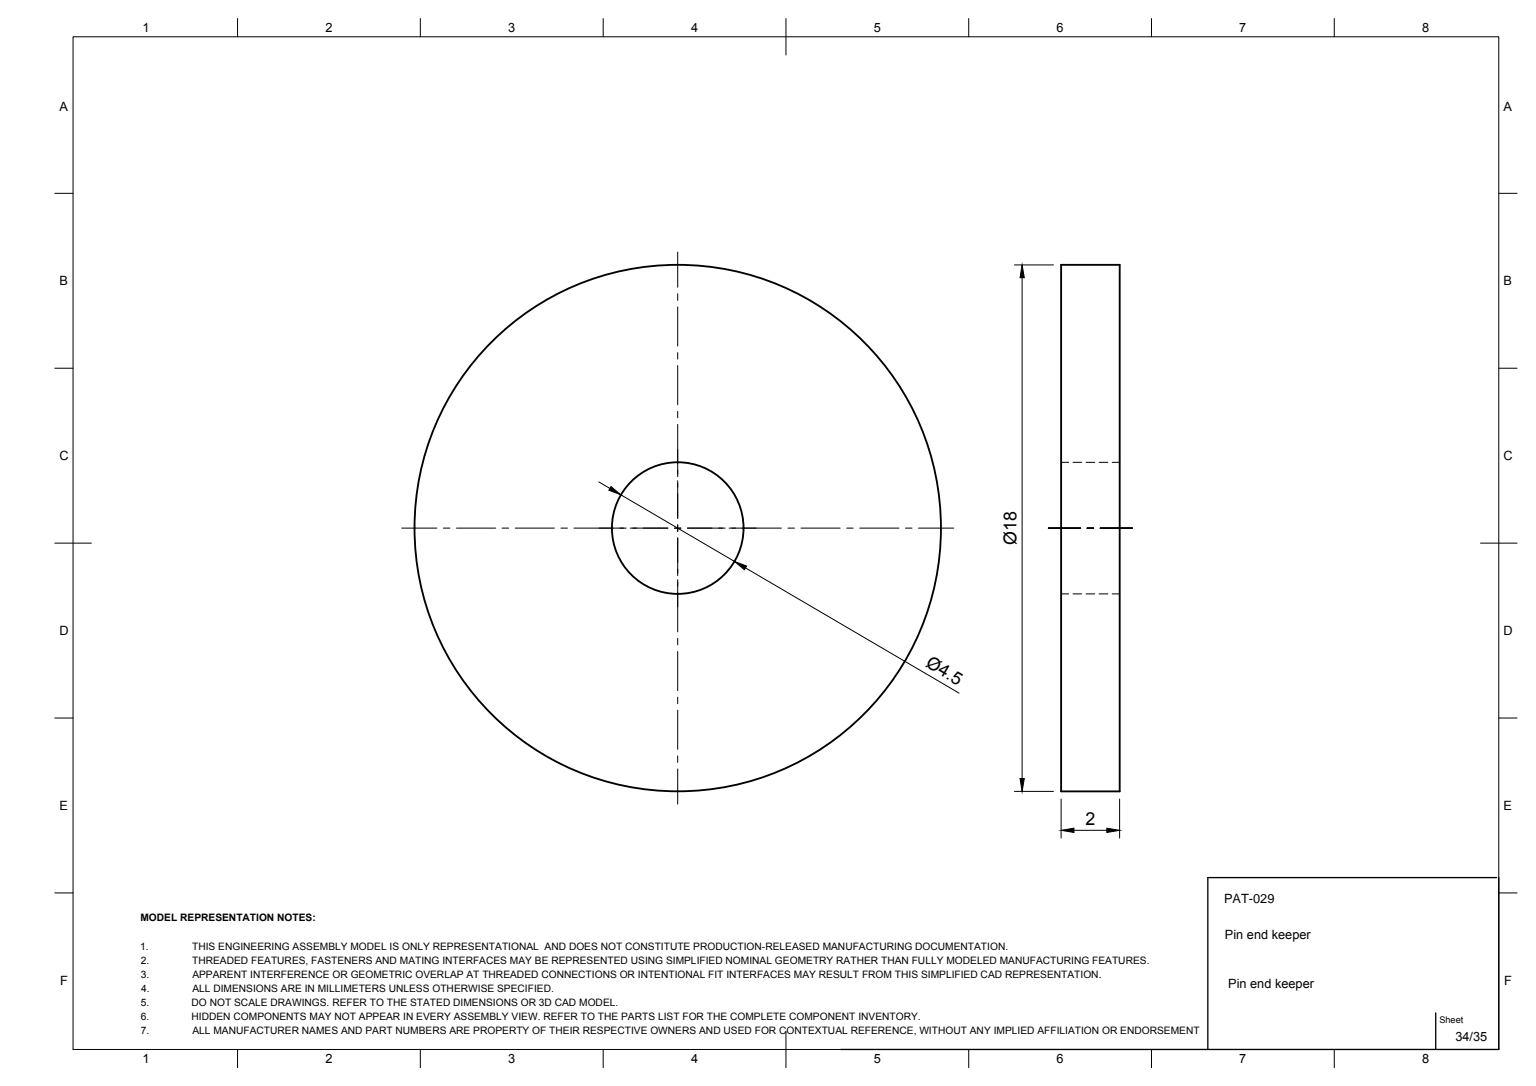
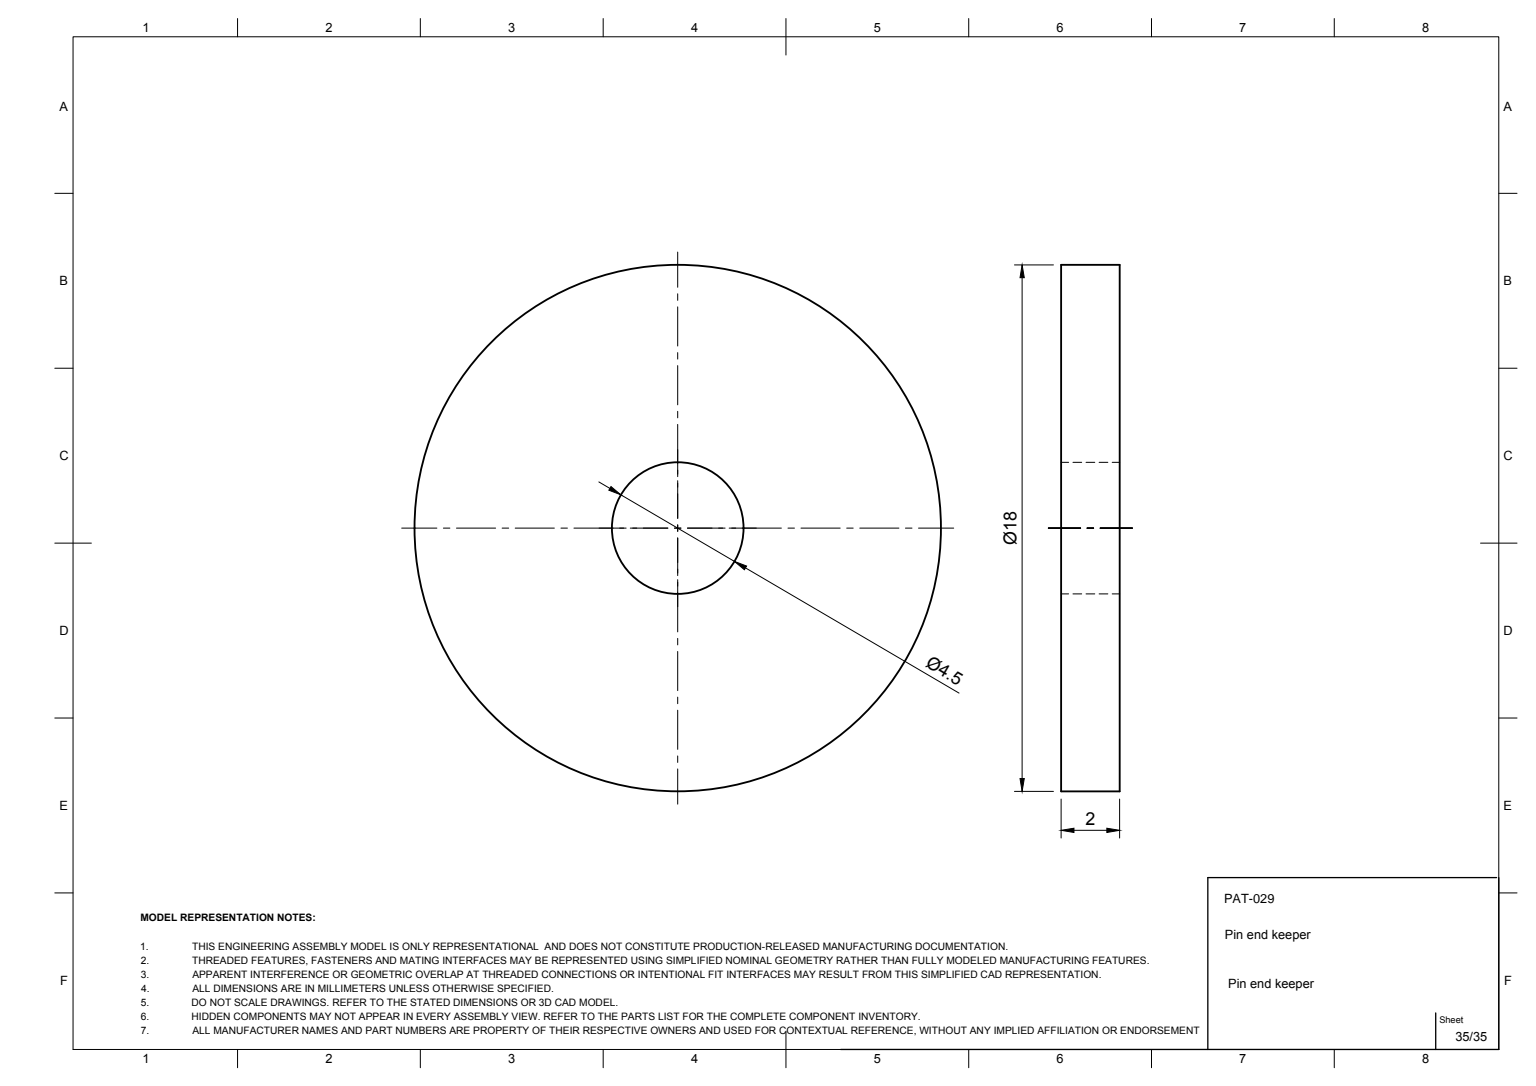
ISO-10303-21;
HEADER;
/* Generated by software containing ST-Developer
 * from STEP Tools, Inc. (www.steptools.com) 
 */

FILE_DESCRIPTION(
/* description */ ('Door-style hinge test fixture with detent'),
/* implementation_level */ '2;1');

FILE_NAME(
/* name */ 'Pin end keeper.step',
/* time_stamp */ '2026-10-28T03:24:57-07:00',
/* author */ (''),
/* organization */ (''),
/* preprocessor_version */ 'ST-DEVELOPER v20.2',
/* originating_system */ 'Autodesk Translation Framework v15.17.0.0',
/* authorisation */ '');

FILE_SCHEMA (('AUTOMOTIVE_DESIGN { 1 0 10303 214 3 1 1 }'));
ENDSEC;

DATA;
#10=MECHANICAL_DESIGN_GEOMETRIC_PRESENTATION_REPRESENTATION('',(#359),#9813);
#288=SHAPE_REPRESENTATION_RELATIONSHIP('SRR','None',#9967,#319);
#319=ADVANCED_BREP_SHAPE_REPRESENTATION('',(#397),#9810);
#359=STYLED_ITEM('',(#10183),#397);
#397=MANIFOLD_SOLID_BREP('Body1',#4792);
#495=FACE_BOUND('',#1307,.T.);
#496=FACE_BOUND('',#1309,.T.);
#648=PLANE('',#5705);
#649=PLANE('',#5706);
#923=FACE_OUTER_BOUND('',#1304,.T.);
#924=FACE_OUTER_BOUND('',#1305,.T.);
#925=FACE_OUTER_BOUND('',#1306,.T.);
#926=FACE_OUTER_BOUND('',#1308,.T.);
#1304=EDGE_LOOP('',(#4293,#4294,#4295,#4296));
#1305=EDGE_LOOP('',(#4297,#4298,#4299,#4300));
#1306=EDGE_LOOP('',(#4301));
#1307=EDGE_LOOP('',(#4302));
#1308=EDGE_LOOP('',(#4303));
#1309=EDGE_LOOP('',(#4304));
#1626=LINE('',#9638,#1946);
#1627=LINE('',#9644,#1947);
#1946=VECTOR('',#7169,0.225);
#1947=VECTOR('',#7176,0.9);
#2205=CIRCLE('',#5700,0.225);
#2206=CIRCLE('',#5701,0.225);
#2207=CIRCLE('',#5703,0.9);
#2208=CIRCLE('',#5704,0.9);
#2592=VERTEX_POINT('',#9635);
#2593=VERTEX_POINT('',#9637);
#2594=VERTEX_POINT('',#9641);
#2595=VERTEX_POINT('',#9643);
#3163=EDGE_CURVE('',#2592,#2592,#2205,.T.);
#3164=EDGE_CURVE('',#2592,#2593,#1626,.T.);
#3165=EDGE_CURVE('',#2593,#2593,#2206,.T.);
#3166=EDGE_CURVE('',#2594,#2594,#2207,.T.);
#3167=EDGE_CURVE('',#2594,#2595,#1627,.T.);
#3168=EDGE_CURVE('',#2595,#2595,#2208,.T.);
#4293=ORIENTED_EDGE('',*,*,#3163,.F.);
#4294=ORIENTED_EDGE('',*,*,#3164,.T.);
#4295=ORIENTED_EDGE('',*,*,#3165,.T.);
#4296=ORIENTED_EDGE('',*,*,#3164,.F.);
#4297=ORIENTED_EDGE('',*,*,#3166,.F.);
#4298=ORIENTED_EDGE('',*,*,#3167,.T.);
#4299=ORIENTED_EDGE('',*,*,#3168,.T.);
#4300=ORIENTED_EDGE('',*,*,#3167,.F.);
#4301=ORIENTED_EDGE('',*,*,#3166,.T.);
#4302=ORIENTED_EDGE('',*,*,#3163,.T.);
#4303=ORIENTED_EDGE('',*,*,#3168,.F.);
#4304=ORIENTED_EDGE('',*,*,#3165,.F.);
#4462=CYLINDRICAL_SURFACE('',#5699,0.225);
#4463=CYLINDRICAL_SURFACE('',#5702,0.9);
#4728=ADVANCED_FACE('',(#923),#4462,.F.);
#4729=ADVANCED_FACE('',(#924),#4463,.T.);
#4730=ADVANCED_FACE('',(#925,#495),#648,.T.);
#4731=ADVANCED_FACE('',(#926,#496),#649,.F.);
#4792=CLOSED_SHELL('',(#4728,#4729,#4730,#4731));
#5698=AXIS2_PLACEMENT_3D('',#9633,#7163,#7164);
#5699=AXIS2_PLACEMENT_3D('',#9634,#7165,#7166);
#5700=AXIS2_PLACEMENT_3D('',#9636,#7167,#7168);
#5701=AXIS2_PLACEMENT_3D('',#9639,#7170,#7171);
#5702=AXIS2_PLACEMENT_3D('',#9640,#7172,#7173);
#5703=AXIS2_PLACEMENT_3D('',#9642,#7174,#7175);
#5704=AXIS2_PLACEMENT_3D('',#9645,#7177,#7178);
#5705=AXIS2_PLACEMENT_3D('',#9646,#7179,#7180);
#5706=AXIS2_PLACEMENT_3D('',#9647,#7181,#7182);
#7163=DIRECTION('axis',(0.,0.,1.));
#7164=DIRECTION('refdir',(1.,0.,0.));
#7165=DIRECTION('center_axis',(0.,0.,1.));
#7166=DIRECTION('ref_axis',(1.,0.,0.));
#7167=DIRECTION('center_axis',(0.,0.,-1.));
#7168=DIRECTION('ref_axis',(1.,0.,0.));
#7169=DIRECTION('',(0.,0.,-1.));
#7170=DIRECTION('center_axis',(0.,0.,-1.));
#7171=DIRECTION('ref_axis',(1.,0.,0.));
#7172=DIRECTION('center_axis',(0.,0.,1.));
#7173=DIRECTION('ref_axis',(1.,0.,0.));
#7174=DIRECTION('center_axis',(0.,0.,1.));
#7175=DIRECTION('ref_axis',(1.,0.,0.));
#7176=DIRECTION('',(0.,0.,-1.));
#7177=DIRECTION('center_axis',(0.,0.,1.));
#7178=DIRECTION('ref_axis',(1.,0.,0.));
#7179=DIRECTION('center_axis',(0.,0.,1.));
#7180=DIRECTION('ref_axis',(1.,0.,0.));
#7181=DIRECTION('center_axis',(0.,0.,1.));
#7182=DIRECTION('ref_axis',(1.,0.,0.));
#9633=CARTESIAN_POINT('',(0.,0.,0.));
#9634=CARTESIAN_POINT('Origin',(0.,0.,1.8));
#9635=CARTESIAN_POINT('',(-0.225,-2.75545529808154E-17,2.));
#9636=CARTESIAN_POINT('Origin',(0.,0.,2.));
#9637=CARTESIAN_POINT('',(-0.225,-2.75545529808154E-17,1.8));
#9638=CARTESIAN_POINT('',(-0.225,-2.75545529808154E-17,1.8));
#9639=CARTESIAN_POINT('Origin',(0.,0.,1.8));
#9640=CARTESIAN_POINT('Origin',(0.,0.,1.8));
#9641=CARTESIAN_POINT('',(-0.9,-1.10218211923262E-16,2.));
#9642=CARTESIAN_POINT('Origin',(0.,0.,2.));
#9643=CARTESIAN_POINT('',(-0.9,-1.10218211923262E-16,1.8));
#9644=CARTESIAN_POINT('',(-0.9,-1.10218211923262E-16,1.8));
#9645=CARTESIAN_POINT('Origin',(0.,0.,1.8));
#9646=CARTESIAN_POINT('Origin',(0.,0.,2.));
#9647=CARTESIAN_POINT('Origin',(0.,0.,1.8));
#9774=UNCERTAINTY_MEASURE_WITH_UNIT(LENGTH_MEASURE(0.001),#9814,
'DISTANCE_ACCURACY_VALUE',
'Maximum model space distance between geometric entities at asserted c
onnectivities');
#9777=UNCERTAINTY_MEASURE_WITH_UNIT(LENGTH_MEASURE(0.001),#9814,
'DISTANCE_ACCURACY_VALUE',
'Maximum model space distance between geometric entities at asserted c
onnectivities');
#9810=(
GEOMETRIC_REPRESENTATION_CONTEXT(3)
GLOBAL_UNCERTAINTY_ASSIGNED_CONTEXT((#9774))
GLOBAL_UNIT_ASSIGNED_CONTEXT((#9814,#9816,#9817))
REPRESENTATION_CONTEXT('','3D')
);
#9813=(
GEOMETRIC_REPRESENTATION_CONTEXT(3)
GLOBAL_UNCERTAINTY_ASSIGNED_CONTEXT((#9777))
GLOBAL_UNIT_ASSIGNED_CONTEXT((#9814,#9816,#9817))
REPRESENTATION_CONTEXT('','3D')
);
#9814=(
LENGTH_UNIT()
NAMED_UNIT(*)
SI_UNIT(.CENTI.,.METRE.)
);
#9816=(
NAMED_UNIT(*)
PLANE_ANGLE_UNIT()
SI_UNIT($,.RADIAN.)
);
#9817=(
NAMED_UNIT(*)
SI_UNIT($,.STERADIAN.)
SOLID_ANGLE_UNIT()
);
#9850=SHAPE_DEFINITION_REPRESENTATION(#9923,#9967);
#9923=PRODUCT_DEFINITION_SHAPE('',$,#10003);
#9967=SHAPE_REPRESENTATION('',(#5698),#9810);
#9970=PRODUCT_DEFINITION_CONTEXT('part definition',#10077,'design');
#10003=PRODUCT_DEFINITION('Pin end keeper','Pin end keeper',#10038,#9970);
#10038=PRODUCT_DEFINITION_FORMATION('',$,#10111);
#10077=APPLICATION_CONTEXT(
'Core Data for Automotive Mechanical Design Process');
#10078=PRODUCT_CONTEXT('part definition',#10077,'mechanical');
#10111=PRODUCT('Pin end keeper','Pin end keeper','Pin end keeper',(#10078));
#10177=COLOUR_RGB('Grey',0.48,0.52,0.57);
#10178=FILL_AREA_STYLE_COLOUR('',#10177);
#10179=FILL_AREA_STYLE('',(#10178));
#10180=SURFACE_STYLE_FILL_AREA(#10179);
#10181=SURFACE_SIDE_STYLE('',(#10180));
#10182=SURFACE_STYLE_USAGE(.BOTH.,#10181);
#10183=PRESENTATION_STYLE_ASSIGNMENT((#10182));
ENDSEC;
END-ISO-10303-21;
